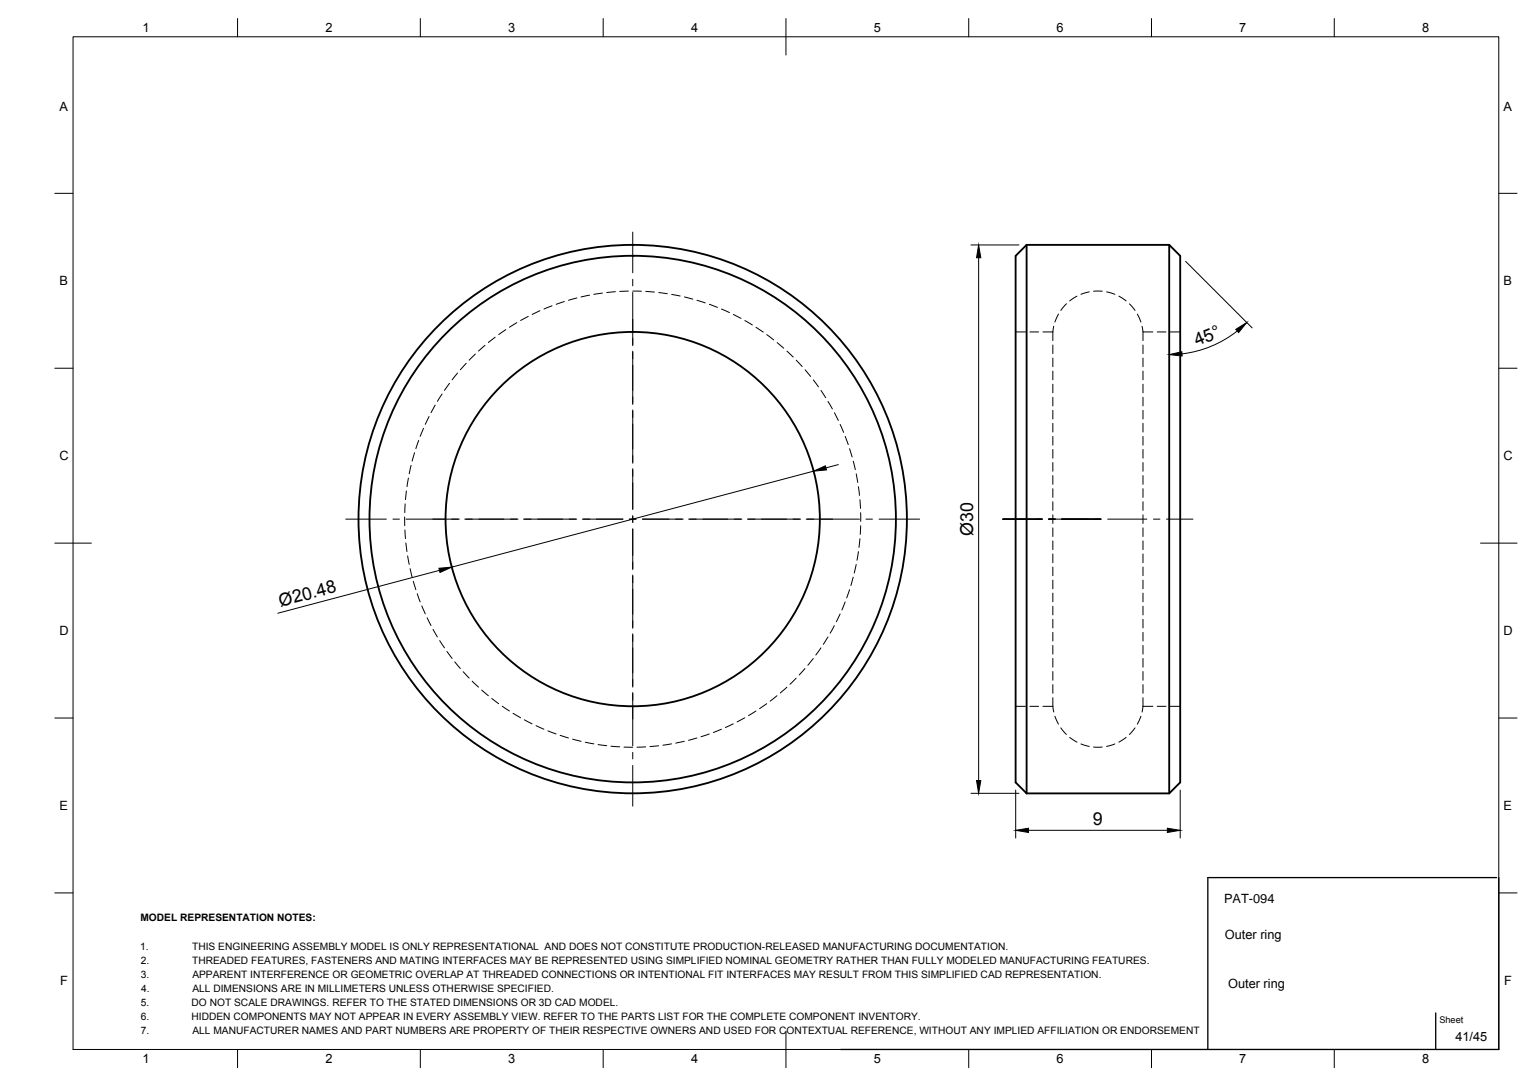
ISO-10303-21;
HEADER;
/* Generated by software containing ST-Developer
 * from STEP Tools, Inc. (www.steptools.com) 
 */

FILE_DESCRIPTION(
/* description */ ('Shaft runout checking stand'),
/* implementation_level */ '2;1');

FILE_NAME(
/* name */ 'Outer ring.step',
/* time_stamp */ '2026-11-02T21:12:33-08:00',
/* author */ (''),
/* organization */ (''),
/* preprocessor_version */ 'ST-DEVELOPER v20.2',
/* originating_system */ 'Autodesk Translation Framework v15.17.0.0',
/* authorisation */ '');

FILE_SCHEMA (('AUTOMOTIVE_DESIGN { 1 0 10303 214 3 1 1 }'));
ENDSEC;

DATA;
#10=MECHANICAL_DESIGN_GEOMETRIC_PRESENTATION_REPRESENTATION('',(#499),#11748);
#28=TOROIDAL_SURFACE('',#7343,1.,0.247676);
#373=CONICAL_SURFACE('',#7354,1.47,0.785398163397449);
#374=CONICAL_SURFACE('',#7358,1.47,0.785398163397449);
#413=SHAPE_REPRESENTATION_RELATIONSHIP('SRR','None',#11965,#456);
#456=ADVANCED_BREP_SHAPE_REPRESENTATION('',(#547),#11741);
#499=STYLED_ITEM('',(#12170),#547);
#547=MANIFOLD_SOLID_BREP('Body1',#6245);
#660=FACE_BOUND('',#1820,.T.);
#661=FACE_BOUND('',#1825,.T.);
#865=CIRCLE('',#7344,1.023815);
#866=CIRCLE('',#7345,1.023815);
#867=CIRCLE('',#7346,0.247676);
#868=CIRCLE('',#7347,1.023815);
#869=CIRCLE('',#7348,1.023815);
#870=CIRCLE('',#7350,1.023815);
#871=CIRCLE('',#7352,1.44);
#872=CIRCLE('',#7353,1.023815);
#873=CIRCLE('',#7355,1.5);
#874=CIRCLE('',#7357,1.5);
#875=CIRCLE('',#7359,1.44);
#1023=CYLINDRICAL_SURFACE('',#7349,1.023815);
#1024=CYLINDRICAL_SURFACE('',#7356,1.5);
#1025=CYLINDRICAL_SURFACE('',#7361,1.023815);
#1351=FACE_OUTER_BOUND('',#1817,.T.);
#1352=FACE_OUTER_BOUND('',#1818,.T.);
#1353=FACE_OUTER_BOUND('',#1819,.T.);
#1354=FACE_OUTER_BOUND('',#1821,.T.);
#1355=FACE_OUTER_BOUND('',#1822,.T.);
#1356=FACE_OUTER_BOUND('',#1823,.T.);
#1357=FACE_OUTER_BOUND('',#1824,.T.);
#1358=FACE_OUTER_BOUND('',#1826,.T.);
#1817=EDGE_LOOP('',(#5388,#5389,#5390,#5391,#5392,#5393));
#1818=EDGE_LOOP('',(#5394,#5395,#5396,#5397,#5398));
#1819=EDGE_LOOP('',(#5399));
#1820=EDGE_LOOP('',(#5400));
#1821=EDGE_LOOP('',(#5401,#5402,#5403,#5404));
#1822=EDGE_LOOP('',(#5405,#5406,#5407,#5408));
#1823=EDGE_LOOP('',(#5409,#5410,#5411,#5412));
#1824=EDGE_LOOP('',(#5413));
#1825=EDGE_LOOP('',(#5414));
#1826=EDGE_LOOP('',(#5415,#5416,#5417,#5418,#5419));
#2335=LINE('',#11060,#2802);
#2336=LINE('',#11069,#2803);
#2337=LINE('',#11073,#2804);
#2338=LINE('',#11077,#2805);
#2339=LINE('',#11080,#2806);
#2802=VECTOR('',#9176,1.023815);
#2803=VECTOR('',#9187,1.47);
#2804=VECTOR('',#9192,1.5);
#2805=VECTOR('',#9197,1.47);
#2806=VECTOR('',#9202,1.023815);
#3248=VERTEX_POINT('',#11048);
#3249=VERTEX_POINT('',#11049);
#3250=VERTEX_POINT('',#11052);
#3251=VERTEX_POINT('',#11054);
#3252=VERTEX_POINT('',#11058);
#3253=VERTEX_POINT('',#11062);
#3254=VERTEX_POINT('',#11064);
#3255=VERTEX_POINT('',#11067);
#3256=VERTEX_POINT('',#11071);
#3257=VERTEX_POINT('',#11075);
#3980=EDGE_CURVE('',#3248,#3249,#865,.T.);
#3981=EDGE_CURVE('',#3249,#3248,#866,.T.);
#3982=EDGE_CURVE('',#3249,#3250,#867,.T.);
#3983=EDGE_CURVE('',#3251,#3250,#868,.T.);
#3984=EDGE_CURVE('',#3250,#3251,#869,.T.);
#3985=EDGE_CURVE('',#3252,#3252,#870,.T.);
#3986=EDGE_CURVE('',#3252,#3251,#2335,.T.);
#3987=EDGE_CURVE('',#3253,#3253,#871,.T.);
#3988=EDGE_CURVE('',#3254,#3254,#872,.T.);
#3989=EDGE_CURVE('',#3255,#3255,#873,.T.);
#3990=EDGE_CURVE('',#3255,#3253,#2336,.T.);
#3991=EDGE_CURVE('',#3256,#3256,#874,.T.);
#3992=EDGE_CURVE('',#3256,#3255,#2337,.T.);
#3993=EDGE_CURVE('',#3257,#3257,#875,.T.);
#3994=EDGE_CURVE('',#3257,#3256,#2338,.T.);
#3995=EDGE_CURVE('',#3248,#3254,#2339,.T.);
#5388=ORIENTED_EDGE('',*,*,#3980,.F.);
#5389=ORIENTED_EDGE('',*,*,#3981,.F.);
#5390=ORIENTED_EDGE('',*,*,#3982,.T.);
#5391=ORIENTED_EDGE('',*,*,#3983,.F.);
#5392=ORIENTED_EDGE('',*,*,#3984,.F.);
#5393=ORIENTED_EDGE('',*,*,#3982,.F.);
#5394=ORIENTED_EDGE('',*,*,#3985,.T.);
#5395=ORIENTED_EDGE('',*,*,#3986,.T.);
#5396=ORIENTED_EDGE('',*,*,#3983,.T.);
#5397=ORIENTED_EDGE('',*,*,#3984,.T.);
#5398=ORIENTED_EDGE('',*,*,#3986,.F.);
#5399=ORIENTED_EDGE('',*,*,#3987,.F.);
#5400=ORIENTED_EDGE('',*,*,#3988,.T.);
#5401=ORIENTED_EDGE('',*,*,#3989,.F.);
#5402=ORIENTED_EDGE('',*,*,#3990,.T.);
#5403=ORIENTED_EDGE('',*,*,#3987,.T.);
#5404=ORIENTED_EDGE('',*,*,#3990,.F.);
#5405=ORIENTED_EDGE('',*,*,#3991,.F.);
#5406=ORIENTED_EDGE('',*,*,#3992,.T.);
#5407=ORIENTED_EDGE('',*,*,#3989,.T.);
#5408=ORIENTED_EDGE('',*,*,#3992,.F.);
#5409=ORIENTED_EDGE('',*,*,#3993,.F.);
#5410=ORIENTED_EDGE('',*,*,#3994,.T.);
#5411=ORIENTED_EDGE('',*,*,#3991,.T.);
#5412=ORIENTED_EDGE('',*,*,#3994,.F.);
#5413=ORIENTED_EDGE('',*,*,#3993,.T.);
#5414=ORIENTED_EDGE('',*,*,#3985,.F.);
#5415=ORIENTED_EDGE('',*,*,#3980,.T.);
#5416=ORIENTED_EDGE('',*,*,#3981,.T.);
#5417=ORIENTED_EDGE('',*,*,#3995,.T.);
#5418=ORIENTED_EDGE('',*,*,#3988,.F.);
#5419=ORIENTED_EDGE('',*,*,#3995,.F.);
#5817=PLANE('',#7351);
#5818=PLANE('',#7360);
#6151=ADVANCED_FACE('',(#1351),#28,.F.);
#6152=ADVANCED_FACE('',(#1352),#1023,.F.);
#6153=ADVANCED_FACE('',(#1353,#660),#5817,.T.);
#6154=ADVANCED_FACE('',(#1354),#373,.T.);
#6155=ADVANCED_FACE('',(#1355),#1024,.T.);
#6156=ADVANCED_FACE('',(#1356),#374,.T.);
#6157=ADVANCED_FACE('',(#1357,#661),#5818,.T.);
#6158=ADVANCED_FACE('',(#1358),#1025,.F.);
#6245=CLOSED_SHELL('',(#6151,#6152,#6153,#6154,#6155,#6156,#6157,#6158));
#7342=AXIS2_PLACEMENT_3D('',#11046,#9158,#9159);
#7343=AXIS2_PLACEMENT_3D('',#11047,#9160,#9161);
#7344=AXIS2_PLACEMENT_3D('',#11050,#9162,#9163);
#7345=AXIS2_PLACEMENT_3D('',#11051,#9164,#9165);
#7346=AXIS2_PLACEMENT_3D('',#11053,#9166,#9167);
#7347=AXIS2_PLACEMENT_3D('',#11055,#9168,#9169);
#7348=AXIS2_PLACEMENT_3D('',#11056,#9170,#9171);
#7349=AXIS2_PLACEMENT_3D('',#11057,#9172,#9173);
#7350=AXIS2_PLACEMENT_3D('',#11059,#9174,#9175);
#7351=AXIS2_PLACEMENT_3D('',#11061,#9177,#9178);
#7352=AXIS2_PLACEMENT_3D('',#11063,#9179,#9180);
#7353=AXIS2_PLACEMENT_3D('',#11065,#9181,#9182);
#7354=AXIS2_PLACEMENT_3D('',#11066,#9183,#9184);
#7355=AXIS2_PLACEMENT_3D('',#11068,#9185,#9186);
#7356=AXIS2_PLACEMENT_3D('',#11070,#9188,#9189);
#7357=AXIS2_PLACEMENT_3D('',#11072,#9190,#9191);
#7358=AXIS2_PLACEMENT_3D('',#11074,#9193,#9194);
#7359=AXIS2_PLACEMENT_3D('',#11076,#9195,#9196);
#7360=AXIS2_PLACEMENT_3D('',#11078,#9198,#9199);
#7361=AXIS2_PLACEMENT_3D('',#11079,#9200,#9201);
#9158=DIRECTION('axis',(0.,0.,1.));
#9159=DIRECTION('refdir',(1.,0.,0.));
#9160=DIRECTION('center_axis',(0.,-1.,0.));
#9161=DIRECTION('ref_axis',(0.,0.,-1.));
#9162=DIRECTION('center_axis',(0.,-1.,0.));
#9163=DIRECTION('ref_axis',(1.,0.,0.));
#9164=DIRECTION('center_axis',(0.,-1.,0.));
#9165=DIRECTION('ref_axis',(1.,0.,0.));
#9166=DIRECTION('center_axis',(1.,0.,1.22464679914735E-16));
#9167=DIRECTION('ref_axis',(-1.22464679914735E-16,0.,1.));
#9168=DIRECTION('center_axis',(0.,1.,0.));
#9169=DIRECTION('ref_axis',(1.,0.,0.));
#9170=DIRECTION('center_axis',(0.,1.,0.));
#9171=DIRECTION('ref_axis',(1.,0.,0.));
#9172=DIRECTION('center_axis',(0.,-1.,0.));
#9173=DIRECTION('ref_axis',(1.,0.,0.));
#9174=DIRECTION('center_axis',(0.,-1.,0.));
#9175=DIRECTION('ref_axis',(1.,0.,0.));
#9176=DIRECTION('',(0.,1.,0.));
#9177=DIRECTION('center_axis',(0.,1.,0.));
#9178=DIRECTION('ref_axis',(0.,0.,1.));
#9179=DIRECTION('center_axis',(0.,-1.,0.));
#9180=DIRECTION('ref_axis',(1.,0.,0.));
#9181=DIRECTION('center_axis',(0.,-1.,0.));
#9182=DIRECTION('ref_axis',(1.,0.,0.));
#9183=DIRECTION('center_axis',(0.,-1.,0.));
#9184=DIRECTION('ref_axis',(1.,0.,0.));
#9185=DIRECTION('center_axis',(0.,-1.,0.));
#9186=DIRECTION('ref_axis',(1.,0.,0.));
#9187=DIRECTION('',(0.707106781186548,0.707106781186547,8.65956056235494E-17));
#9188=DIRECTION('center_axis',(0.,-1.,0.));
#9189=DIRECTION('ref_axis',(1.,0.,0.));
#9190=DIRECTION('center_axis',(0.,-1.,0.));
#9191=DIRECTION('ref_axis',(1.,0.,0.));
#9192=DIRECTION('',(0.,1.,0.));
#9193=DIRECTION('center_axis',(0.,1.,0.));
#9194=DIRECTION('ref_axis',(1.,0.,0.));
#9195=DIRECTION('center_axis',(0.,-1.,0.));
#9196=DIRECTION('ref_axis',(1.,0.,0.));
#9197=DIRECTION('',(-0.707106781186548,0.707106781186547,-8.65956056235494E-17));
#9198=DIRECTION('center_axis',(0.,-1.,0.));
#9199=DIRECTION('ref_axis',(0.,0.,-1.));
#9200=DIRECTION('center_axis',(0.,-1.,0.));
#9201=DIRECTION('ref_axis',(1.,0.,0.));
#9202=DIRECTION('',(0.,1.,0.));
#11046=CARTESIAN_POINT('',(0.,0.,0.));
#11047=CARTESIAN_POINT('Origin',(0.,0.,0.));
#11048=CARTESIAN_POINT('',(-1.023815,0.246528389340863,-1.25381176266905E-16));
#11049=CARTESIAN_POINT('',(-1.25381176266905E-16,0.246528389340863,1.023815));
#11050=CARTESIAN_POINT('Origin',(0.,0.246528389340863,0.));
#11051=CARTESIAN_POINT('Origin',(0.,0.246528389340863,0.));
#11052=CARTESIAN_POINT('',(-1.25381176266905E-16,-0.246528389340863,1.023815));
#11053=CARTESIAN_POINT('Origin',(-1.22464679914735E-16,0.,1.));
#11054=CARTESIAN_POINT('',(-1.023815,-0.246528389340863,1.25381176266905E-16));
#11055=CARTESIAN_POINT('Origin',(0.,-0.246528389340863,0.));
#11056=CARTESIAN_POINT('Origin',(0.,-0.246528389340863,0.));
#11057=CARTESIAN_POINT('Origin',(0.,0.,0.));
#11058=CARTESIAN_POINT('',(-1.023815,-0.45,-1.25381176266905E-16));
#11059=CARTESIAN_POINT('Origin',(0.,-0.45,0.));
#11060=CARTESIAN_POINT('',(-1.023815,0.,-1.25381176266905E-16));
#11061=CARTESIAN_POINT('Origin',(1.44,0.45,0.));
#11062=CARTESIAN_POINT('',(-1.44,0.45,-1.76349139077219E-16));
#11063=CARTESIAN_POINT('Origin',(0.,0.45,0.));
#11064=CARTESIAN_POINT('',(-1.023815,0.45,-1.25381176266905E-16));
#11065=CARTESIAN_POINT('Origin',(0.,0.45,0.));
#11066=CARTESIAN_POINT('Origin',(0.,0.42,0.));
#11067=CARTESIAN_POINT('',(-1.5,0.39,-1.83697019872103E-16));
#11068=CARTESIAN_POINT('Origin',(0.,0.39,0.));
#11069=CARTESIAN_POINT('',(-1.47,0.42,-1.80023079474661E-16));
#11070=CARTESIAN_POINT('Origin',(0.,0.,0.));
#11071=CARTESIAN_POINT('',(-1.5,-0.39,-1.83697019872103E-16));
#11072=CARTESIAN_POINT('Origin',(0.,-0.39,0.));
#11073=CARTESIAN_POINT('',(-1.5,0.,-1.83697019872103E-16));
#11074=CARTESIAN_POINT('Origin',(0.,-0.42,0.));
#11075=CARTESIAN_POINT('',(-1.44,-0.45,-1.76349139077219E-16));
#11076=CARTESIAN_POINT('Origin',(0.,-0.45,0.));
#11077=CARTESIAN_POINT('',(-1.47,-0.42,-1.80023079474661E-16));
#11078=CARTESIAN_POINT('Origin',(1.023815,-0.45,0.));
#11079=CARTESIAN_POINT('Origin',(0.,0.,0.));
#11080=CARTESIAN_POINT('',(-1.023815,0.,-1.25381176266905E-16));
#11692=UNCERTAINTY_MEASURE_WITH_UNIT(LENGTH_MEASURE(0.001),#11749,
'DISTANCE_ACCURACY_VALUE',
'Maximum model space distance between geometric entities at asserted c
onnectivities');
#11699=UNCERTAINTY_MEASURE_WITH_UNIT(LENGTH_MEASURE(0.001),#11749,
'DISTANCE_ACCURACY_VALUE',
'Maximum model space distance between geometric entities at asserted c
onnectivities');
#11741=(
GEOMETRIC_REPRESENTATION_CONTEXT(3)
GLOBAL_UNCERTAINTY_ASSIGNED_CONTEXT((#11692))
GLOBAL_UNIT_ASSIGNED_CONTEXT((#11749,#11751,#11752))
REPRESENTATION_CONTEXT('','3D')
);
#11748=(
GEOMETRIC_REPRESENTATION_CONTEXT(3)
GLOBAL_UNCERTAINTY_ASSIGNED_CONTEXT((#11699))
GLOBAL_UNIT_ASSIGNED_CONTEXT((#11749,#11751,#11752))
REPRESENTATION_CONTEXT('','3D')
);
#11749=(
LENGTH_UNIT()
NAMED_UNIT(*)
SI_UNIT(.CENTI.,.METRE.)
);
#11751=(
NAMED_UNIT(*)
PLANE_ANGLE_UNIT()
SI_UNIT($,.RADIAN.)
);
#11752=(
NAMED_UNIT(*)
SI_UNIT($,.STERADIAN.)
SOLID_ANGLE_UNIT()
);
#11794=SHAPE_DEFINITION_REPRESENTATION(#11902,#11965);
#11902=PRODUCT_DEFINITION_SHAPE('',$,#12014);
#11965=SHAPE_REPRESENTATION('',(#7342),#11741);
#11972=PRODUCT_DEFINITION_CONTEXT('part definition',#12118,'design');
#12014=PRODUCT_DEFINITION('Outer ring','Outer ring',#12062,#11972);
#12062=PRODUCT_DEFINITION_FORMATION('',$,#12161);
#12118=APPLICATION_CONTEXT(
'Core Data for Automotive Mechanical Design Process');
#12119=PRODUCT_CONTEXT('part definition',#12118,'mechanical');
#12161=PRODUCT('Outer ring','Outer ring','Outer ring',(#12119));
#12170=PRESENTATION_STYLE_ASSIGNMENT((#12175));
#12175=SURFACE_STYLE_USAGE(.BOTH.,#12180);
#12180=SURFACE_SIDE_STYLE('',(#12185));
#12185=SURFACE_STYLE_FILL_AREA(#12190);
#12190=FILL_AREA_STYLE('CAD Library Painted - Steel gray',(#12195));
#12195=FILL_AREA_STYLE_COLOUR('CAD Library Painted - Steel gray',#12200);
#12200=COLOUR_RGB('CAD Library Painted - Steel gray',0.592156862745098,
0.631372549019608,0.67843137254902);
ENDSEC;
END-ISO-10303-21;
